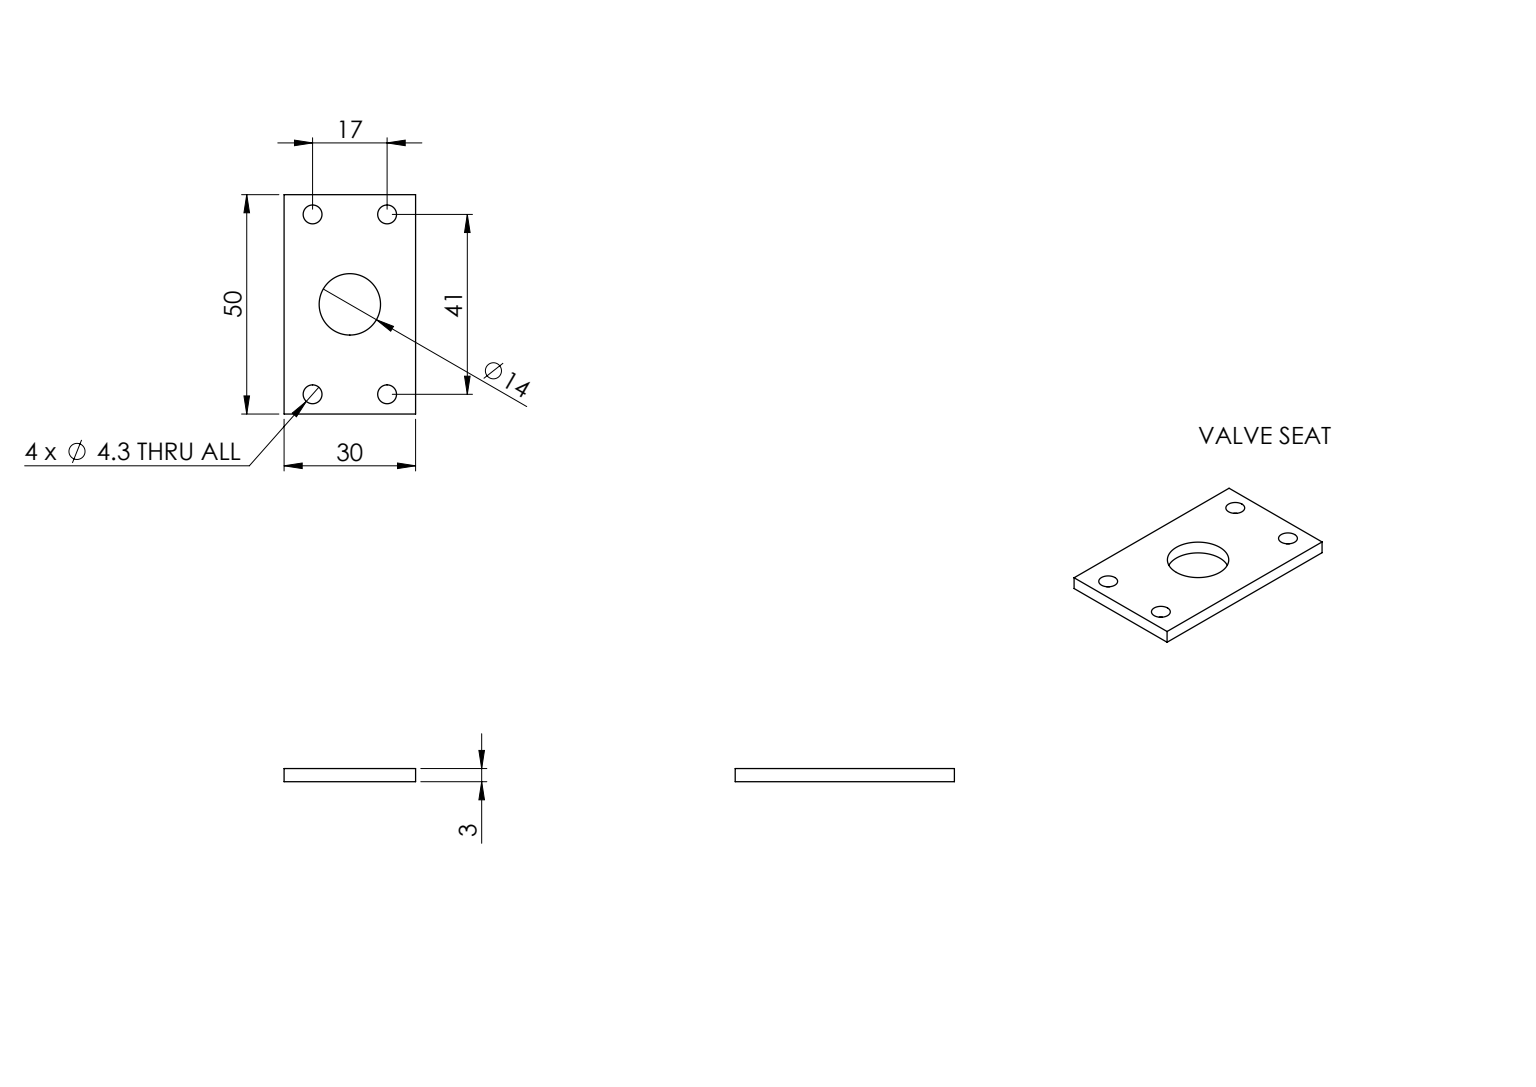
ISO-10303-21;
HEADER;
FILE_DESCRIPTION (('STEP AP214'),
    '1' );
FILE_NAME ('valve seat.step',
    '2026-10-25T16:39:07',
    ( '' ),
    ( '' ),
    'SwSTEP 2.0',
    'SolidWorks 2026',
    '' );
FILE_SCHEMA (( 'AUTOMOTIVE_DESIGN' ));
ENDSEC;

DATA;
#13=VERTEX_POINT ( 'NONE', #16013 ) ;
#121=CARTESIAN_POINT ( 'NONE',  ( 8.500000000000001776, 13.00000000000000178, -20.49999999999999645 ) ) ;
#128=DIRECTION ( 'NONE',  ( -1.000000000000000000, -0.000000000000000000, -0.000000000000000000 ) ) ;
#265=CARTESIAN_POINT ( 'NONE',  ( 8.673617379884035472E-15, 13.00000000000000178, 3.469446951953614189E-15 ) ) ;
#291=ORIENTED_EDGE ( 'NONE', *, *, #12084, .T. ) ;
#295=( NAMED_UNIT ( * ) PLANE_ANGLE_UNIT ( ) SI_UNIT ( $, .RADIAN. ) );
#319=EDGE_CURVE ( 'NONE', #18210, #10649, #7063, .T. ) ;
#321=LINE ( 'NONE', #17400, #16399 ) ;
#436=CARTESIAN_POINT ( 'NONE',  ( 14.99999999999999822, 13.00000000000000178, -25.00000000000000355 ) ) ;
#493=AXIS2_PLACEMENT_3D ( 'NONE', #9507, #8120, #16856 ) ;
#497=FACE_OUTER_BOUND ( 'NONE', #16040, .T. ) ;
#498=ORIENTED_EDGE ( 'NONE', *, *, #5184, .F. ) ;
#538=DIRECTION ( 'NONE',  ( -1.000000000000000000, 0.000000000000000000, 0.000000000000000000 ) ) ;
#543=AXIS2_PLACEMENT_3D ( 'NONE', #16285, #14984, #3573 ) ;
#557=( NAMED_UNIT ( * ) SI_UNIT ( $, .STERADIAN. ) SOLID_ANGLE_UNIT ( ) );
#636=FACE_OUTER_BOUND ( 'NONE', #10821, .T. ) ;
#646=VERTEX_POINT ( 'NONE', #1074 ) ;
#653=ORIENTED_EDGE ( 'NONE', *, *, #13216, .F. ) ;
#734=ADVANCED_FACE ( 'NONE', ( #5775 ), #14125, .F. ) ;
#775=EDGE_LOOP ( 'NONE', ( #10453, #6606, #13929, #968 ) ) ;
#797=DIRECTION ( 'NONE',  ( 0.000000000000000000, 0.000000000000000000, 1.000000000000000000 ) ) ;
#806=ORIENTED_EDGE ( 'NONE', *, *, #9638, .F. ) ;
#822=AXIS2_PLACEMENT_3D ( 'NONE', #16795, #15489, #1027 ) ;
#885=AXIS2_PLACEMENT_3D ( 'NONE', #7012, #8412, #13804 ) ;
#927=AXIS2_PLACEMENT_3D ( 'NONE', #1459, #7089, #2934 ) ;
#968=ORIENTED_EDGE ( 'NONE', *, *, #11920, .T. ) ;
#979=DIRECTION ( 'NONE',  ( -0.000000000000000000, -0.000000000000000000, 1.000000000000000000 ) ) ;
#991=VECTOR ( 'NONE', #7879, 1000.000000000000000 ) ;
#999=CARTESIAN_POINT ( 'NONE',  ( -15.00000000000000178, 13.00000000000000178, 24.99999999999999645 ) ) ;
#1027=DIRECTION ( 'NONE',  ( 0.000000000000000000, 0.000000000000000000, 1.000000000000000000 ) ) ;
#1074=CARTESIAN_POINT ( 'NONE',  ( 8.499999999999994671, 13.00000000000000178, 18.35000000000000142 ) ) ;
#1077=VECTOR ( 'NONE', #14132, 1000.000000000000000 ) ;
#1182=CARTESIAN_POINT ( 'NONE',  ( 8.500000000000001776, 10.00000000000000000, -20.49999999999999645 ) ) ;
#1189=CYLINDRICAL_SURFACE ( 'NONE', #927, 2.149999999999995470 ) ;
#1217=ORIENTED_EDGE ( 'NONE', *, *, #2834, .F. ) ;
#1266=ORIENTED_EDGE ( 'NONE', *, *, #2716, .F. ) ;
#1275=DIRECTION ( 'NONE',  ( -0.000000000000000000, 1.000000000000000000, -0.000000000000000000 ) ) ;
#1360=DIRECTION ( 'NONE',  ( 0.000000000000000000, 0.000000000000000000, 1.000000000000000000 ) ) ;
#1384=ADVANCED_FACE ( 'NONE', ( #11965 ), #2159, .F. ) ;
#1454=AXIS2_PLACEMENT_3D ( 'NONE', #1182, #11165, #2395 ) ;
#1459=CARTESIAN_POINT ( 'NONE',  ( 8.499999999999994671, 15.00000000000000178, 20.49999999999999645 ) ) ;
#1550=AXIS2_PLACEMENT_3D ( 'NONE', #5822, #8419, #10170 ) ;
#1564=CIRCLE ( 'NONE', #16681, 2.149999999999999023 ) ;
#1648=FACE_OUTER_BOUND ( 'NONE', #6847, .T. ) ;
#1684=DIRECTION ( 'NONE',  ( -0.000000000000000000, -0.000000000000000000, 1.000000000000000000 ) ) ;
#1737=CYLINDRICAL_SURFACE ( 'NONE', #18184, 2.149999999999995470 ) ;
#1770=ORIENTED_EDGE ( 'NONE', *, *, #6248, .F. ) ;
#1813=EDGE_LOOP ( 'NONE', ( #2295, #17707 ) ) ;
#1838=MECHANICAL_DESIGN_GEOMETRIC_PRESENTATION_REPRESENTATION('',(#15169),#7739);
#1880=FACE_OUTER_BOUND ( 'NONE', #2980, .T. ) ;
#1917=EDGE_CURVE ( 'NONE', #2431, #13322, #9840, .T. ) ;
#1959=VERTEX_POINT ( 'NONE', #6006 ) ;
#1975=DIRECTION ( 'NONE',  ( 0.000000000000000000, 0.000000000000000000, 1.000000000000000000 ) ) ;
#2030=ADVANCED_FACE ( 'NONE', ( #15844 ), #16037, .F. ) ;
#2053=VECTOR ( 'NONE', #4732, 1000.000000000000000 ) ;
#2080=PLANE ( 'NONE',  #12045 ) ;
#2099=EDGE_CURVE ( 'NONE', #13, #16617, #1564, .T. ) ;
#2103=FACE_BOUND ( 'NONE', #1813, .T. ) ;
#2159=PLANE ( 'NONE',  #10421 ) ;
#2184=EDGE_LOOP ( 'NONE', ( #18223, #5378, #6453, #10869 ) ) ;
#2195=FACE_BOUND ( 'NONE', #2494, .T. ) ;
#2204=VERTEX_POINT ( 'NONE', #17186 ) ;
#2206=CYLINDRICAL_SURFACE ( 'NONE', #8950, 2.149999999999995470 ) ;
#2208=DIRECTION ( 'NONE',  ( -0.000000000000000000, 1.000000000000000000, -0.000000000000000000 ) ) ;
#2217=PLANE ( 'NONE',  #16276 ) ;
#2218=MANIFOLD_SOLID_BREP ( 'M4 Clearance Hole1', #2906 ) ;
#2246=ORIENTED_EDGE ( 'NONE', *, *, #11807, .F. ) ;
#2254=LINE ( 'NONE', #9092, #991 ) ;
#2268=EDGE_LOOP ( 'NONE', ( #13436, #12204, #9696, #9451 ) ) ;
#2269=VERTEX_POINT ( 'NONE', #3262 ) ;
#2272=ORIENTED_EDGE ( 'NONE', *, *, #13752, .T. ) ;
#2295=ORIENTED_EDGE ( 'NONE', *, *, #15819, .F. ) ;
#2298=CIRCLE ( 'NONE', #9082, 2.149999999999999023 ) ;
#2306=ADVANCED_FACE ( 'NONE', ( #1880 ), #14577, .F. ) ;
#2314=VECTOR ( 'NONE', #15723, 1000.000000000000000 ) ;
#2375=CARTESIAN_POINT ( 'NONE',  ( 0.000000000000000000, 13.00000000000000178, 0.000000000000000000 ) ) ;
#2395=DIRECTION ( 'NONE',  ( 0.000000000000000000, 0.000000000000000000, 1.000000000000000000 ) ) ;
#2431=VERTEX_POINT ( 'NONE', #16518 ) ;
#2492=CARTESIAN_POINT ( 'NONE',  ( 8.673617379884035472E-15, 13.00000000000000178, 3.469446951953614189E-15 ) ) ;
#2494=EDGE_LOOP ( 'NONE', ( #9062, #15099 ) ) ;
#2539=ORIENTED_EDGE ( 'NONE', *, *, #17953, .T. ) ;
#2610=ORIENTED_EDGE ( 'NONE', *, *, #3037, .T. ) ;
#2617=VECTOR ( 'NONE', #12733, 1000.000000000000000 ) ;
#2619=EDGE_LOOP ( 'NONE', ( #9085, #6999 ) ) ;
#2630=ORIENTED_EDGE ( 'NONE', *, *, #4559, .F. ) ;
#2716=EDGE_CURVE ( 'NONE', #5029, #13163, #321, .T. ) ;
#2755=CARTESIAN_POINT ( 'NONE',  ( 8.673617379884035472E-15, 10.00000000000000000, -6.999999999999996447 ) ) ;
#2778=ORIENTED_EDGE ( 'NONE', *, *, #9638, .T. ) ;
#2780=CARTESIAN_POINT ( 'NONE',  ( -15.00000000000000178, 13.00000000000000178, 24.99999999999999645 ) ) ;
#2825=DIRECTION ( 'NONE',  ( 0.000000000000000000, 0.000000000000000000, -1.000000000000000000 ) ) ;
#2834=EDGE_CURVE ( 'NONE', #7772, #3408, #17185, .T. ) ;
#2855=CIRCLE ( 'NONE', #493, 2.149999999999995470 ) ;
#2896=VERTEX_POINT ( 'NONE', #11770 ) ;
#2906=CLOSED_SHELL ( 'NONE', ( #734, #2306, #10402, #14951, #12373, #4515, #10108, #15058, #1384, #7566, #10663, #2030, #4792, #17733, #3930, #18078 ) ) ;
#2923=DIRECTION ( 'NONE',  ( 1.000000000000000000, 0.000000000000000000, 0.000000000000000000 ) ) ;
#2934=DIRECTION ( 'NONE',  ( 0.000000000000000000, 0.000000000000000000, 1.000000000000000000 ) ) ;
#2980=EDGE_LOOP ( 'NONE', ( #16300, #15846, #10901, #18032 ) ) ;
#2998=DIRECTION ( 'NONE',  ( -0.000000000000000000, 1.000000000000000000, -0.000000000000000000 ) ) ;
#3037=EDGE_CURVE ( 'NONE', #2269, #2431, #8332, .T. ) ;
#3044=DIRECTION ( 'NONE',  ( 0.000000000000000000, 0.000000000000000000, 1.000000000000000000 ) ) ;
#3146=( NAMED_UNIT ( * ) SI_UNIT ( $, .STERADIAN. ) SOLID_ANGLE_UNIT ( ) );
#3155=ORIENTED_EDGE ( 'NONE', *, *, #15116, .F. ) ;
#3163=EDGE_CURVE ( 'NONE', #13322, #2431, #10104, .T. ) ;
#3233=DIRECTION ( 'NONE',  ( 0.000000000000000000, 0.000000000000000000, -1.000000000000000000 ) ) ;
#3262=CARTESIAN_POINT ( 'NONE',  ( -8.500000000000010658, 10.00000000000000000, 22.64999999999998437 ) ) ;
#3317=EDGE_LOOP ( 'NONE', ( #16483, #11941, #1266, #4428 ) ) ;
#3329=DIRECTION ( 'NONE',  ( -0.000000000000000000, -1.000000000000000000, -0.000000000000000000 ) ) ;
#3336=DIRECTION ( 'NONE',  ( 0.000000000000000000, 0.000000000000000000, -1.000000000000000000 ) ) ;
#3374=CARTESIAN_POINT ( 'NONE',  ( 8.673617379884035472E-15, 13.00000000000000178, 3.469446951953614189E-15 ) ) ;
#3408=VERTEX_POINT ( 'NONE', #6099 ) ;
#3460=CARTESIAN_POINT ( 'NONE',  ( -8.500000000000005329, 13.00000000000000178, -22.64999999999999147 ) ) ;
#3490=PRODUCT_CONTEXT ( 'NONE', #10071, 'mechanical' ) ;
#3549=CIRCLE ( 'NONE', #885, 7.000000000000000000 ) ;
#3573=DIRECTION ( 'NONE',  ( 0.000000000000000000, 0.000000000000000000, 1.000000000000000000 ) ) ;
#3624=DIRECTION ( 'NONE',  ( -0.000000000000000000, 1.000000000000000000, -0.000000000000000000 ) ) ;
#3641=CARTESIAN_POINT ( 'NONE',  ( -15.00000000000000178, 13.00000000000000178, 24.99999999999999645 ) ) ;
#3642=AXIS2_PLACEMENT_3D ( 'NONE', #16523, #10485, #16338 ) ;
#3668=FACE_OUTER_BOUND ( 'NONE', #14133, .T. ) ;
#3714=PLANE ( 'NONE',  #3642 ) ;
#3795=CARTESIAN_POINT ( 'NONE',  ( -8.500000000000010658, 15.00000000000000178, 22.64999999999998437 ) ) ;
#3870=ORIENTED_EDGE ( 'NONE', *, *, #1917, .T. ) ;
#3930=ADVANCED_FACE ( 'NONE', ( #9230 ), #2206, .F. ) ;
#3990=CIRCLE ( 'NONE', #12545, 2.149999999999995470 ) ;
#4020=CARTESIAN_POINT ( 'NONE',  ( 8.500000000000001776, 10.00000000000000000, -20.49999999999999645 ) ) ;
#4274=ORIENTED_EDGE ( 'NONE', *, *, #10452, .F. ) ;
#4275=ORIENTED_EDGE ( 'NONE', *, *, #13245, .F. ) ;
#4290=DIRECTION ( 'NONE',  ( 0.000000000000000000, 0.000000000000000000, 1.000000000000000000 ) ) ;
#4327=ORIENTED_EDGE ( 'NONE', *, *, #15402, .T. ) ;
#4416=VERTEX_POINT ( 'NONE', #17565 ) ;
#4428=ORIENTED_EDGE ( 'NONE', *, *, #16591, .T. ) ;
#4500=LINE ( 'NONE', #10140, #18114 ) ;
#4515=ADVANCED_FACE ( 'NONE', ( #17923, #10847, #13536, #4837, #6409, #7605 ), #3714, .T. ) ;
#4524=ORIENTED_EDGE ( 'NONE', *, *, #12834, .F. ) ;
#4559=EDGE_CURVE ( 'NONE', #2896, #7772, #2254, .T. ) ;
#4578=VERTEX_POINT ( 'NONE', #16141 ) ;
#4594=CARTESIAN_POINT ( 'NONE',  ( -8.500000000000010658, 15.00000000000000178, 20.49999999999998934 ) ) ;
#4626=ORIENTED_EDGE ( 'NONE', *, *, #14416, .F. ) ;
#4670=VECTOR ( 'NONE', #17689, 1000.000000000000000 ) ;
#4709=LINE ( 'NONE', #10072, #18017 ) ;
#4732=DIRECTION ( 'NONE',  ( -0.000000000000000000, -1.000000000000000000, -0.000000000000000000 ) ) ;
#4792=ADVANCED_FACE ( 'NONE', ( #12934 ), #1737, .F. ) ;
#4797=AXIS2_PLACEMENT_3D ( 'NONE', #17933, #16813, #10950 ) ;
#4837=FACE_OUTER_BOUND ( 'NONE', #16452, .T. ) ;
#4865=FACE_OUTER_BOUND ( 'NONE', #2268, .T. ) ;
#4889=CARTESIAN_POINT ( 'NONE',  ( 8.500000000000001776, 13.00000000000000178, -20.49999999999999645 ) ) ;
#4916=VECTOR ( 'NONE', #9948, 1000.000000000000000 ) ;
#4951=AXIS2_PLACEMENT_3D ( 'NONE', #4889, #15936, #3233 ) ;
#4963=DIRECTION ( 'NONE',  ( 0.000000000000000000, 0.000000000000000000, 1.000000000000000000 ) ) ;
#5029=VERTEX_POINT ( 'NONE', #436 ) ;
#5114=AXIS2_PLACEMENT_3D ( 'NONE', #16334, #3624, #16243 ) ;
#5122=VERTEX_POINT ( 'NONE', #17701 ) ;
#5158=DIRECTION ( 'NONE',  ( 0.000000000000000000, 0.000000000000000000, 1.000000000000000000 ) ) ;
#5184=EDGE_CURVE ( 'NONE', #13, #646, #14632, .T. ) ;
#5187=ORIENTED_EDGE ( 'NONE', *, *, #17953, .F. ) ;
#5202=ORIENTED_EDGE ( 'NONE', *, *, #5184, .T. ) ;
#5228=LINE ( 'NONE', #16563, #2617 ) ;
#5283=ORIENTED_EDGE ( 'NONE', *, *, #3163, .T. ) ;
#5306=SHAPE_REPRESENTATION ( 'valve seat', ( #16940 ), #7446 ) ;
#5327=AXIS2_PLACEMENT_3D ( 'NONE', #2780, #5541, #11549 ) ;
#5378=ORIENTED_EDGE ( 'NONE', *, *, #8416, .T. ) ;
#5461=CARTESIAN_POINT ( 'NONE',  ( -8.500000000000005329, 10.00000000000000000, -20.49999999999999645 ) ) ;
#5524=CARTESIAN_POINT ( 'NONE',  ( -8.500000000000005329, 15.00000000000000178, -18.35000000000000142 ) ) ;
#5541=DIRECTION ( 'NONE',  ( 1.000000000000000000, -0.000000000000000000, 0.000000000000000000 ) ) ;
#5573=AXIS2_PLACEMENT_3D ( 'NONE', #121, #9853, #2825 ) ;
#5601=DIRECTION ( 'NONE',  ( -0.000000000000000000, 1.000000000000000000, -0.000000000000000000 ) ) ;
#5638=VECTOR ( 'NONE', #14121, 1000.000000000000000 ) ;
#5664=VERTEX_POINT ( 'NONE', #13474 ) ;
#5697=CARTESIAN_POINT ( 'NONE',  ( -15.00000000000000178, 13.00000000000000178, 24.99999999999999645 ) ) ;
#5712=CARTESIAN_POINT ( 'NONE',  ( 14.99999999999999822, 10.00000000000000000, 24.99999999999999645 ) ) ;
#5715=MECHANICAL_DESIGN_GEOMETRIC_PRESENTATION_REPRESENTATION('',(#6603),#14001);
#5775=FACE_OUTER_BOUND ( 'NONE', #6105, .T. ) ;
#5822=CARTESIAN_POINT ( 'NONE',  ( -8.500000000000010658, 13.00000000000000178, 20.49999999999998934 ) ) ;
#5847=CIRCLE ( 'NONE', #16526, 2.149999999999995470 ) ;
#5861=CARTESIAN_POINT ( 'NONE',  ( -8.500000000000010658, 10.00000000000000000, 20.49999999999998934 ) ) ;
#6006=CARTESIAN_POINT ( 'NONE',  ( 8.500000000000001776, 10.00000000000000000, -22.64999999999999503 ) ) ;
#6014=VECTOR ( 'NONE', #6757, 1000.000000000000000 ) ;
#6049=LINE ( 'NONE', #6337, #6760 ) ;
#6083=VECTOR ( 'NONE', #2923, 1000.000000000000000 ) ;
#6092=ORIENTED_EDGE ( 'NONE', *, *, #2099, .T. ) ;
#6099=CARTESIAN_POINT ( 'NONE',  ( -15.00000000000000178, 10.00000000000000000, 24.99999999999999645 ) ) ;
#6105=EDGE_LOOP ( 'NONE', ( #13504, #17153, #806, #7661 ) ) ;
#6117=LINE ( 'NONE', #10281, #2053 ) ;
#6131=AXIS2_PLACEMENT_3D ( 'NONE', #17103, #2998, #17483 ) ;
#6187=LINE ( 'NONE', #13226, #12611 ) ;
#6204=EDGE_LOOP ( 'NONE', ( #6356, #2272 ) ) ;
#6207=EDGE_LOOP ( 'NONE', ( #498, #4275, #11171, #12765 ) ) ;
#6248=EDGE_CURVE ( 'NONE', #3408, #17590, #18338, .T. ) ;
#6274=COLOUR_RGB ( '',0.8941176470588234615, 0.8941176470588234615, 0.8941176470588234615 ) ;
#6275=CARTESIAN_POINT ( 'NONE',  ( -15.00000000000000178, 10.00000000000000000, -25.00000000000000355 ) ) ;
#6337=CARTESIAN_POINT ( 'NONE',  ( 8.500000000000001776, 15.00000000000000178, -22.64999999999999147 ) ) ;
#6356=ORIENTED_EDGE ( 'NONE', *, *, #13216, .T. ) ;
#6409=FACE_BOUND ( 'NONE', #2619, .T. ) ;
#6428=DIRECTION ( 'NONE',  ( 1.000000000000000000, 0.000000000000000000, 0.000000000000000000 ) ) ;
#6438=FACE_BOUND ( 'NONE', #9250, .T. ) ;
#6443=CARTESIAN_POINT ( 'NONE',  ( 14.99999999999999822, 13.00000000000000178, 24.99999999999999645 ) ) ;
#6453=ORIENTED_EDGE ( 'NONE', *, *, #13386, .T. ) ;
#6457=DIRECTION ( 'NONE',  ( 0.000000000000000000, 0.000000000000000000, 1.000000000000000000 ) ) ;
#6491=PRODUCT_DEFINITION_CONTEXT ( 'detailed design', #6987, 'design' ) ;
#6603=STYLED_ITEM('',(#18424),#2218);
#6606=ORIENTED_EDGE ( 'NONE', *, *, #16591, .F. ) ;
#6626=CARTESIAN_POINT ( 'NONE',  ( 14.99999999999999822, 13.00000000000000178, 24.99999999999999645 ) ) ;
#6687=VERTEX_POINT ( 'NONE', #15880 ) ;
#6757=DIRECTION ( 'NONE',  ( -0.000000000000000000, 1.000000000000000000, -0.000000000000000000 ) ) ;
#6760=VECTOR ( 'NONE', #17489, 1000.000000000000000 ) ;
#6811=EDGE_CURVE ( 'NONE', #5122, #4416, #12334, .T. ) ;
#6814=ORIENTED_EDGE ( 'NONE', *, *, #9269, .F. ) ;
#6847=EDGE_LOOP ( 'NONE', ( #9333, #4524, #12672, #13933 ) ) ;
#6902=ORIENTED_EDGE ( 'NONE', *, *, #3163, .F. ) ;
#6947=UNCERTAINTY_MEASURE_WITH_UNIT (LENGTH_MEASURE( 1.000000000000000082E-05 ), #10172, 'distance_accuracy_value', 'NONE');
#6987=APPLICATION_CONTEXT ( 'automotive_design' ) ;
#6999=ORIENTED_EDGE ( 'NONE', *, *, #14791, .T. ) ;
#7012=CARTESIAN_POINT ( 'NONE',  ( 8.673617379884035472E-15, 10.00000000000000000, 3.469446951953614189E-15 ) ) ;
#7034=ORIENTED_EDGE ( 'NONE', *, *, #11920, .F. ) ;
#7063=CIRCLE ( 'NONE', #17155, 2.149999999999995470 ) ;
#7089=DIRECTION ( 'NONE',  ( -0.000000000000000000, 1.000000000000000000, -0.000000000000000000 ) ) ;
#7097=DIRECTION ( 'NONE',  ( 0.000000000000000000, 0.000000000000000000, 1.000000000000000000 ) ) ;
#7115=EDGE_LOOP ( 'NONE', ( #4626, #3155, #16825, #10215 ) ) ;
#7132=AXIS2_PLACEMENT_3D ( 'NONE', #16380, #14811, #797 ) ;
#7396=SURFACE_STYLE_FILL_AREA ( #13055 ) ;
#7446=( GEOMETRIC_REPRESENTATION_CONTEXT ( 3 ) GLOBAL_UNCERTAINTY_ASSIGNED_CONTEXT ( ( #18290 ) ) GLOBAL_UNIT_ASSIGNED_CONTEXT ( ( #7674, #10364, #3146 ) ) REPRESENTATION_CONTEXT ( 'NONE', 'WORKASPACE' ) );
#7464=VERTEX_POINT ( 'NONE', #16696 ) ;
#7477=DIRECTION ( 'NONE',  ( 0.000000000000000000, 0.000000000000000000, -1.000000000000000000 ) ) ;
#7566=ADVANCED_FACE ( 'NONE', ( #1648 ), #10159, .F. ) ;
#7568=VECTOR ( 'NONE', #14280, 1000.000000000000000 ) ;
#7605=FACE_BOUND ( 'NONE', #15364, .T. ) ;
#7641=CYLINDRICAL_SURFACE ( 'NONE', #7132, 2.149999999999995470 ) ;
#7655=CYLINDRICAL_SURFACE ( 'NONE', #12104, 2.149999999999995470 ) ;
#7661=ORIENTED_EDGE ( 'NONE', *, *, #11348, .F. ) ;
#7674=( LENGTH_UNIT ( ) NAMED_UNIT ( * ) SI_UNIT ( .MILLI., .METRE. ) );
#7739=( GEOMETRIC_REPRESENTATION_CONTEXT ( 3 ) GLOBAL_UNCERTAINTY_ASSIGNED_CONTEXT ( ( #6947 ) ) GLOBAL_UNIT_ASSIGNED_CONTEXT ( ( #10172, #12958, #557 ) ) REPRESENTATION_CONTEXT ( 'NONE', 'WORKASPACE' ) );
#7772=VERTEX_POINT ( 'NONE', #6275 ) ;
#7778=AXIS2_PLACEMENT_3D ( 'NONE', #265, #3329, #15941 ) ;
#7805=CARTESIAN_POINT ( 'NONE',  ( -8.500000000000005329, 13.00000000000000178, -18.35000000000000142 ) ) ;
#7836=ADVANCED_BREP_SHAPE_REPRESENTATION ( '', ( #2218, #16940 ), #7446 ) ;
#7853=VERTEX_POINT ( 'NONE', #999 ) ;
#7872=CIRCLE ( 'NONE', #17070, 2.149999999999995470 ) ;
#7879=DIRECTION ( 'NONE',  ( -1.000000000000000000, -0.000000000000000000, -0.000000000000000000 ) ) ;
#7902=CIRCLE ( 'NONE', #10856, 2.149999999999995470 ) ;
#7932=DIRECTION ( 'NONE',  ( -0.000000000000000000, 1.000000000000000000, -0.000000000000000000 ) ) ;
#7960=DIRECTION ( 'NONE',  ( 0.000000000000000000, -1.000000000000000000, 0.000000000000000000 ) ) ;
#7969=EDGE_LOOP ( 'NONE', ( #9908, #15671 ) ) ;
#8120=DIRECTION ( 'NONE',  ( 0.000000000000000000, -1.000000000000000000, 0.000000000000000000 ) ) ;
#8124=VERTEX_POINT ( 'NONE', #2755 ) ;
#8145=CARTESIAN_POINT ( 'NONE',  ( -15.00000000000000178, 13.00000000000000178, -25.00000000000000355 ) ) ;
#8276=AXIS2_PLACEMENT_3D ( 'NONE', #11417, #17205, #8456 ) ;
#8332=LINE ( 'NONE', #3795, #6014 ) ;
#8405=ORIENTED_EDGE ( 'NONE', *, *, #11348, .T. ) ;
#8412=DIRECTION ( 'NONE',  ( 0.000000000000000000, 1.000000000000000000, 0.000000000000000000 ) ) ;
#8416=EDGE_CURVE ( 'NONE', #5122, #5664, #12783, .T. ) ;
#8419=DIRECTION ( 'NONE',  ( 0.000000000000000000, -1.000000000000000000, 0.000000000000000000 ) ) ;
#8456=DIRECTION ( 'NONE',  ( 0.000000000000000000, 0.000000000000000000, 1.000000000000000000 ) ) ;
#8686=SURFACE_SIDE_STYLE ('',( #7396 ) ) ;
#8706=EDGE_CURVE ( 'NONE', #11774, #646, #3990, .T. ) ;
#8707=CARTESIAN_POINT ( 'NONE',  ( -15.00000000000000178, 10.00000000000000000, 24.99999999999999645 ) ) ;
#8752=DIRECTION ( 'NONE',  ( -0.000000000000000000, 1.000000000000000000, -0.000000000000000000 ) ) ;
#8790=CIRCLE ( 'NONE', #822, 2.149999999999999023 ) ;
#8950=AXIS2_PLACEMENT_3D ( 'NONE', #10433, #11916, #4963 ) ;
#8965=LINE ( 'NONE', #15809, #1077 ) ;
#9024=CARTESIAN_POINT ( 'NONE',  ( 0.000000000000000000, 0.000000000000000000, 0.000000000000000000 ) ) ;
#9041=CARTESIAN_POINT ( 'NONE',  ( -8.500000000000005329, 13.00000000000000178, -20.49999999999999645 ) ) ;
#9058=DIRECTION ( 'NONE',  ( 0.000000000000000000, 0.000000000000000000, -1.000000000000000000 ) ) ;
#9062=ORIENTED_EDGE ( 'NONE', *, *, #8706, .T. ) ;
#9082=AXIS2_PLACEMENT_3D ( 'NONE', #4020, #12729, #4290 ) ;
#9085=ORIENTED_EDGE ( 'NONE', *, *, #10452, .T. ) ;
#9092=CARTESIAN_POINT ( 'NONE',  ( -15.00000000000000178, 10.00000000000000000, -25.00000000000000355 ) ) ;
#9151=CARTESIAN_POINT ( 'NONE',  ( 8.499999999999994671, 13.00000000000000178, 20.49999999999999645 ) ) ;
#9163=VECTOR ( 'NONE', #11369, 1000.000000000000000 ) ;
#9170=EDGE_CURVE ( 'NONE', #646, #11774, #7872, .T. ) ;
#9197=EDGE_CURVE ( 'NONE', #17590, #2896, #6187, .T. ) ;
#9230=FACE_OUTER_BOUND ( 'NONE', #7115, .T. ) ;
#9239=PRODUCT_DEFINITION_FORMATION_WITH_SPECIFIED_SOURCE ( 'ANY', '', #13293, .NOT_KNOWN. ) ;
#9250=EDGE_LOOP ( 'NONE', ( #3870, #5283 ) ) ;
#9265=EDGE_CURVE ( 'NONE', #13163, #7772, #8965, .T. ) ;
#9269=EDGE_CURVE ( 'NONE', #7853, #18081, #17031, .T. ) ;
#9288=DIRECTION ( 'NONE',  ( 0.000000000000000000, 0.000000000000000000, -1.000000000000000000 ) ) ;
#9333=ORIENTED_EDGE ( 'NONE', *, *, #2834, .T. ) ;
#9396=CARTESIAN_POINT ( 'NONE',  ( 8.500000000000001776, 15.00000000000000178, -18.35000000000000142 ) ) ;
#9451=ORIENTED_EDGE ( 'NONE', *, *, #9269, .T. ) ;
#9463=ORIENTED_EDGE ( 'NONE', *, *, #6248, .T. ) ;
#9507=CARTESIAN_POINT ( 'NONE',  ( -8.500000000000005329, 13.00000000000000178, -20.49999999999999645 ) ) ;
#9622=EDGE_LOOP ( 'NONE', ( #10639, #4327 ) ) ;
#9638=EDGE_CURVE ( 'NONE', #10649, #18210, #2855, .T. ) ;
#9696=ORIENTED_EDGE ( 'NONE', *, *, #10179, .T. ) ;
#9840=CIRCLE ( 'NONE', #18172, 2.149999999999995470 ) ;
#9853=DIRECTION ( 'NONE',  ( 0.000000000000000000, -1.000000000000000000, 0.000000000000000000 ) ) ;
#9874=FACE_OUTER_BOUND ( 'NONE', #6207, .T. ) ;
#9882=DIRECTION ( 'NONE',  ( -0.000000000000000000, 1.000000000000000000, -0.000000000000000000 ) ) ;
#9908=ORIENTED_EDGE ( 'NONE', *, *, #15116, .T. ) ;
#9924=VERTEX_POINT ( 'NONE', #16006 ) ;
#9948=DIRECTION ( 'NONE',  ( 1.000000000000000000, 0.000000000000000000, 0.000000000000000000 ) ) ;
#10023=CYLINDRICAL_SURFACE ( 'NONE', #6131, 2.149999999999995470 ) ;
#10071=APPLICATION_CONTEXT ( 'automotive_design' ) ;
#10072=CARTESIAN_POINT ( 'NONE',  ( 8.673617379884035472E-15, 13.00000000000000178, -6.999999999999996447 ) ) ;
#10104=CIRCLE ( 'NONE', #1550, 2.149999999999995470 ) ;
#10108=ADVANCED_FACE ( 'NONE', ( #13757, #16461, #2195, #6438, #4865, #2103 ), #14981, .F. ) ;
#10140=CARTESIAN_POINT ( 'NONE',  ( -8.500000000000010658, 15.00000000000000178, 18.34999999999999432 ) ) ;
#10159=PLANE ( 'NONE',  #5327 ) ;
#10170=DIRECTION ( 'NONE',  ( 0.000000000000000000, 0.000000000000000000, -1.000000000000000000 ) ) ;
#10172=( LENGTH_UNIT ( ) NAMED_UNIT ( * ) SI_UNIT ( .MILLI., .METRE. ) );
#10179=EDGE_CURVE ( 'NONE', #13163, #7853, #13659, .T. ) ;
#10191=( NAMED_UNIT ( * ) SI_UNIT ( $, .STERADIAN. ) SOLID_ANGLE_UNIT ( ) );
#10214=EDGE_CURVE ( 'NONE', #1959, #9924, #2298, .T. ) ;
#10215=ORIENTED_EDGE ( 'NONE', *, *, #10971, .F. ) ;
#10259=DIRECTION ( 'NONE',  ( 0.000000000000000000, 0.000000000000000000, 1.000000000000000000 ) ) ;
#10281=CARTESIAN_POINT ( 'NONE',  ( -15.00000000000000178, 13.00000000000000178, 24.99999999999999645 ) ) ;
#10363=CARTESIAN_POINT ( 'NONE',  ( -8.500000000000010658, 13.00000000000000178, 20.49999999999998934 ) ) ;
#10364=( NAMED_UNIT ( * ) PLANE_ANGLE_UNIT ( ) SI_UNIT ( $, .RADIAN. ) );
#10402=ADVANCED_FACE ( 'NONE', ( #15985 ), #10023, .F. ) ;
#10421=AXIS2_PLACEMENT_3D ( 'NONE', #16064, #1975, #13357 ) ;
#10433=CARTESIAN_POINT ( 'NONE',  ( 8.500000000000001776, 15.00000000000000178, -20.49999999999999645 ) ) ;
#10452=EDGE_CURVE ( 'NONE', #2269, #2204, #7902, .T. ) ;
#10453=ORIENTED_EDGE ( 'NONE', *, *, #9197, .T. ) ;
#10476=PRODUCT_DEFINITION_SHAPE ( 'NONE', 'NONE',  #16042 ) ;
#10485=DIRECTION ( 'NONE',  ( 0.000000000000000000, -1.000000000000000000, 0.000000000000000000 ) ) ;
#10515=DIRECTION ( 'NONE',  ( 0.000000000000000000, -0.000000000000000000, -1.000000000000000000 ) ) ;
#10540=EDGE_LOOP ( 'NONE', ( #17062, #5202, #13491, #18303 ) ) ;
#10591=CIRCLE ( 'NONE', #543, 7.000000000000000000 ) ;
#10609=LINE ( 'NONE', #6626, #16838 ) ;
#10639=ORIENTED_EDGE ( 'NONE', *, *, #11807, .T. ) ;
#10649=VERTEX_POINT ( 'NONE', #7805 ) ;
#10663=ADVANCED_FACE ( 'NONE', ( #12247 ), #2080, .F. ) ;
#10821=EDGE_LOOP ( 'NONE', ( #14972, #2539, #12113, #14563 ) ) ;
#10847=FACE_BOUND ( 'NONE', #7969, .T. ) ;
#10856=AXIS2_PLACEMENT_3D ( 'NONE', #5861, #11694, #17199 ) ;
#10869=ORIENTED_EDGE ( 'NONE', *, *, #15402, .F. ) ;
#10901=ORIENTED_EDGE ( 'NONE', *, *, #12084, .F. ) ;
#10929=DIRECTION ( 'NONE',  ( 0.000000000000000000, 0.000000000000000000, -1.000000000000000000 ) ) ;
#10950=DIRECTION ( 'NONE',  ( 0.000000000000000000, 0.000000000000000000, 1.000000000000000000 ) ) ;
#10971=EDGE_CURVE ( 'NONE', #7464, #16667, #18313, .T. ) ;
#11106=DIRECTION ( 'NONE',  ( -0.000000000000000000, 1.000000000000000000, -0.000000000000000000 ) ) ;
#11162=CIRCLE ( 'NONE', #15079, 2.149999999999995470 ) ;
#11165=DIRECTION ( 'NONE',  ( -0.000000000000000000, 1.000000000000000000, -0.000000000000000000 ) ) ;
#11171=ORIENTED_EDGE ( 'NONE', *, *, #15380, .T. ) ;
#11343=EDGE_CURVE ( 'NONE', #18081, #5029, #12751, .T. ) ;
#11348=EDGE_CURVE ( 'NONE', #4578, #10649, #15631, .T. ) ;
#11369=DIRECTION ( 'NONE',  ( -0.000000000000000000, 1.000000000000000000, -0.000000000000000000 ) ) ;
#11417=CARTESIAN_POINT ( 'NONE',  ( -8.500000000000005329, 15.00000000000000178, -20.49999999999999645 ) ) ;
#11418=DIRECTION ( 'NONE',  ( 0.000000000000000000, 0.000000000000000000, 1.000000000000000000 ) ) ;
#11435=CARTESIAN_POINT ( 'NONE',  ( 14.99999999999999822, 13.00000000000000178, 24.99999999999999645 ) ) ;
#11454=CARTESIAN_POINT ( 'NONE',  ( -8.500000000000010658, 10.00000000000000000, 20.49999999999998934 ) ) ;
#11476=CIRCLE ( 'NONE', #5573, 2.149999999999995470 ) ;
#11508=CARTESIAN_POINT ( 'NONE',  ( 8.499999999999994671, 10.00000000000000000, 22.64999999999999503 ) ) ;
#11549=DIRECTION ( 'NONE',  ( 0.000000000000000000, 0.000000000000000000, -1.000000000000000000 ) ) ;
#11550=DIRECTION ( 'NONE',  ( -0.000000000000000000, 1.000000000000000000, -0.000000000000000000 ) ) ;
#11655=CARTESIAN_POINT ( 'NONE',  ( 8.499999999999994671, 10.00000000000000000, 20.49999999999999645 ) ) ;
#11661=SHAPE_REPRESENTATION_RELATIONSHIP ( 'NONE' , 'NONE' ,  #5306, #7836 ) ;
#11694=DIRECTION ( 'NONE',  ( -0.000000000000000000, 1.000000000000000000, -0.000000000000000000 ) ) ;
#11770=CARTESIAN_POINT ( 'NONE',  ( 14.99999999999999822, 10.00000000000000000, -25.00000000000000355 ) ) ;
#11774=VERTEX_POINT ( 'NONE', #15164 ) ;
#11807=EDGE_CURVE ( 'NONE', #8124, #4416, #10591, .T. ) ;
#11812=CIRCLE ( 'NONE', #15480, 7.000000000000000000 ) ;
#11863=EDGE_CURVE ( 'NONE', #9924, #16667, #11995, .T. ) ;
#11916=DIRECTION ( 'NONE',  ( -0.000000000000000000, 1.000000000000000000, -0.000000000000000000 ) ) ;
#11920=EDGE_CURVE ( 'NONE', #18081, #17590, #10609, .T. ) ;
#11927=EDGE_CURVE ( 'NONE', #6687, #18210, #5228, .T. ) ;
#11929=CARTESIAN_POINT ( 'NONE',  ( -8.500000000000010658, 15.00000000000000178, 20.49999999999998934 ) ) ;
#11941=ORIENTED_EDGE ( 'NONE', *, *, #9265, .F. ) ;
#11965=FACE_OUTER_BOUND ( 'NONE', #3317, .T. ) ;
#11977=DIRECTION ( 'NONE',  ( -1.000000000000000000, 0.000000000000000000, -0.000000000000000000 ) ) ;
#11995=LINE ( 'NONE', #9396, #4670 ) ;
#12037=ORIENTED_EDGE ( 'NONE', *, *, #6811, .T. ) ;
#12045=AXIS2_PLACEMENT_3D ( 'NONE', #3641, #9288, #11977 ) ;
#12084=EDGE_CURVE ( 'NONE', #16667, #7464, #11476, .T. ) ;
#12104=AXIS2_PLACEMENT_3D ( 'NONE', #11929, #7932, #5158 ) ;
#12113=ORIENTED_EDGE ( 'NONE', *, *, #1917, .F. ) ;
#12118=ORIENTED_EDGE ( 'NONE', *, *, #10971, .T. ) ;
#12177=DIRECTION ( 'NONE',  ( 0.000000000000000000, -1.000000000000000000, 0.000000000000000000 ) ) ;
#12204=ORIENTED_EDGE ( 'NONE', *, *, #2716, .T. ) ;
#12247=FACE_OUTER_BOUND ( 'NONE', #13076, .T. ) ;
#12271=DIRECTION ( 'NONE',  ( -0.000000000000000000, -1.000000000000000000, -0.000000000000000000 ) ) ;
#12334=LINE ( 'NONE', #13064, #7568 ) ;
#12373=ADVANCED_FACE ( 'NONE', ( #497 ), #14693, .F. ) ;
#12425=ORIENTED_EDGE ( 'NONE', *, *, #319, .F. ) ;
#12545=AXIS2_PLACEMENT_3D ( 'NONE', #16700, #7960, #10929 ) ;
#12590=CARTESIAN_POINT ( 'NONE',  ( -8.500000000000010658, 13.00000000000000178, 18.34999999999999432 ) ) ;
#12611=VECTOR ( 'NONE', #9058, 1000.000000000000000 ) ;
#12672=ORIENTED_EDGE ( 'NONE', *, *, #10179, .F. ) ;
#12677=AXIS2_PLACEMENT_3D ( 'NONE', #3374, #16265, #17765 ) ;
#12729=DIRECTION ( 'NONE',  ( -0.000000000000000000, 1.000000000000000000, -0.000000000000000000 ) ) ;
#12733=DIRECTION ( 'NONE',  ( -0.000000000000000000, 1.000000000000000000, -0.000000000000000000 ) ) ;
#12751=LINE ( 'NONE', #11435, #2314 ) ;
#12765=ORIENTED_EDGE ( 'NONE', *, *, #9170, .F. ) ;
#12771=LINE ( 'NONE', #16881, #9163 ) ;
#12783=CIRCLE ( 'NONE', #4797, 7.000000000000000000 ) ;
#12797=ORIENTED_EDGE ( 'NONE', *, *, #9197, .F. ) ;
#12834=EDGE_CURVE ( 'NONE', #7853, #3408, #6117, .T. ) ;
#12934=FACE_OUTER_BOUND ( 'NONE', #17644, .T. ) ;
#12958=( NAMED_UNIT ( * ) PLANE_ANGLE_UNIT ( ) SI_UNIT ( $, .RADIAN. ) );
#12980=( LENGTH_UNIT ( ) NAMED_UNIT ( * ) SI_UNIT ( .MILLI., .METRE. ) );
#13055=FILL_AREA_STYLE ('',( #15755 ) ) ;
#13064=CARTESIAN_POINT ( 'NONE',  ( 9.530870139287183087E-15, 13.00000000000000178, 7.000000000000003553 ) ) ;
#13076=EDGE_LOOP ( 'NONE', ( #9463, #7034, #6814, #16578 ) ) ;
#13091=CARTESIAN_POINT ( 'NONE',  ( 14.99999999999999822, 13.00000000000000178, -25.00000000000000355 ) ) ;
#13163=VERTEX_POINT ( 'NONE', #8145 ) ;
#13216=EDGE_CURVE ( 'NONE', #4578, #6687, #11162, .T. ) ;
#13226=CARTESIAN_POINT ( 'NONE',  ( 14.99999999999999822, 10.00000000000000000, 24.99999999999999645 ) ) ;
#13239=SURFACE_STYLE_USAGE ( .BOTH. , #8686 ) ;
#13245=EDGE_CURVE ( 'NONE', #16617, #13, #8790, .T. ) ;
#13293=PRODUCT ( 'valve seat', 'valve seat', '', ( #3490 ) ) ;
#13322=VERTEX_POINT ( 'NONE', #12590 ) ;
#13357=DIRECTION ( 'NONE',  ( 1.000000000000000000, 0.000000000000000000, -0.000000000000000000 ) ) ;
#13386=EDGE_CURVE ( 'NONE', #5664, #8124, #4709, .T. ) ;
#13391=CARTESIAN_POINT ( 'NONE',  ( -15.00000000000000178, 13.00000000000000178, 24.99999999999999645 ) ) ;
#13436=ORIENTED_EDGE ( 'NONE', *, *, #11343, .T. ) ;
#13474=CARTESIAN_POINT ( 'NONE',  ( 8.673617379884035472E-15, 13.00000000000000178, -6.999999999999996447 ) ) ;
#13491=ORIENTED_EDGE ( 'NONE', *, *, #8706, .F. ) ;
#13504=ORIENTED_EDGE ( 'NONE', *, *, #13752, .F. ) ;
#13536=FACE_BOUND ( 'NONE', #9622, .T. ) ;
#13557=DIRECTION ( 'NONE',  ( 0.000000000000000000, 0.000000000000000000, 1.000000000000000000 ) ) ;
#13659=LINE ( 'NONE', #13391, #16206 ) ;
#13752=EDGE_CURVE ( 'NONE', #6687, #4578, #5847, .T. ) ;
#13757=FACE_BOUND ( 'NONE', #17327, .T. ) ;
#13804=DIRECTION ( 'NONE',  ( 0.000000000000000000, 0.000000000000000000, 1.000000000000000000 ) ) ;
#13928=ORIENTED_EDGE ( 'NONE', *, *, #319, .T. ) ;
#13929=ORIENTED_EDGE ( 'NONE', *, *, #11343, .F. ) ;
#13933=ORIENTED_EDGE ( 'NONE', *, *, #9265, .T. ) ;
#14001=( GEOMETRIC_REPRESENTATION_CONTEXT ( 3 ) GLOBAL_UNCERTAINTY_ASSIGNED_CONTEXT ( ( #15289 ) ) GLOBAL_UNIT_ASSIGNED_CONTEXT ( ( #12980, #295, #10191 ) ) REPRESENTATION_CONTEXT ( 'NONE', 'WORKASPACE' ) );
#14121=DIRECTION ( 'NONE',  ( -0.000000000000000000, -1.000000000000000000, -0.000000000000000000 ) ) ;
#14125=CYLINDRICAL_SURFACE ( 'NONE', #8276, 2.149999999999995470 ) ;
#14126=CARTESIAN_POINT ( 'NONE',  ( -8.500000000000005329, 10.00000000000000000, -20.49999999999999645 ) ) ;
#14132=DIRECTION ( 'NONE',  ( -0.000000000000000000, -1.000000000000000000, -0.000000000000000000 ) ) ;
#14133=EDGE_LOOP ( 'NONE', ( #17444, #653, #8405, #12425 ) ) ;
#14134=CARTESIAN_POINT ( 'NONE',  ( -15.00000000000000178, 10.00000000000000000, 24.99999999999999645 ) ) ;
#14280=DIRECTION ( 'NONE',  ( -0.000000000000000000, -1.000000000000000000, -0.000000000000000000 ) ) ;
#14363=PRESENTATION_STYLE_ASSIGNMENT (( #13239 ) ) ;
#14416=EDGE_CURVE ( 'NONE', #1959, #7464, #6049, .T. ) ;
#14563=ORIENTED_EDGE ( 'NONE', *, *, #3037, .F. ) ;
#14577=CYLINDRICAL_SURFACE ( 'NONE', #5114, 2.149999999999995470 ) ;
#14632=LINE ( 'NONE', #14917, #16397 ) ;
#14693=CYLINDRICAL_SURFACE ( 'NONE', #12677, 7.000000000000000000 ) ;
#14791=EDGE_CURVE ( 'NONE', #2204, #2269, #17162, .T. ) ;
#14811=DIRECTION ( 'NONE',  ( -0.000000000000000000, 1.000000000000000000, -0.000000000000000000 ) ) ;
#14907=DIRECTION ( 'NONE',  ( 0.000000000000000000, 0.000000000000000000, -1.000000000000000000 ) ) ;
#14917=CARTESIAN_POINT ( 'NONE',  ( 8.499999999999994671, 15.00000000000000178, 18.35000000000000142 ) ) ;
#14924=FACE_OUTER_BOUND ( 'NONE', #775, .T. ) ;
#14951=ADVANCED_FACE ( 'NONE', ( #636 ), #7655, .F. ) ;
#14972=ORIENTED_EDGE ( 'NONE', *, *, #14791, .F. ) ;
#14981=PLANE ( 'NONE',  #15029 ) ;
#14984=DIRECTION ( 'NONE',  ( 0.000000000000000000, 1.000000000000000000, 0.000000000000000000 ) ) ;
#15005=CARTESIAN_POINT ( 'NONE',  ( 14.99999999999999822, 13.00000000000000178, 24.99999999999999645 ) ) ;
#15029=AXIS2_PLACEMENT_3D ( 'NONE', #2375, #12177, #10515 ) ;
#15058=ADVANCED_FACE ( 'NONE', ( #14924 ), #2217, .F. ) ;
#15077=AXIS2_PLACEMENT_3D ( 'NONE', #11454, #11550, #3044 ) ;
#15079=AXIS2_PLACEMENT_3D ( 'NONE', #5461, #11106, #16886 ) ;
#15099=ORIENTED_EDGE ( 'NONE', *, *, #9170, .T. ) ;
#15116=EDGE_CURVE ( 'NONE', #9924, #1959, #16567, .T. ) ;
#15164=CARTESIAN_POINT ( 'NONE',  ( 8.499999999999994671, 13.00000000000000178, 22.64999999999999147 ) ) ;
#15169=STYLED_ITEM ( 'NONE', ( #14363 ), #7836 ) ;
#15177=VECTOR ( 'NONE', #1684, 1000.000000000000000 ) ;
#15289=UNCERTAINTY_MEASURE_WITH_UNIT (LENGTH_MEASURE( 1.000000000000000082E-05 ), #12980, 'distance_accuracy_value', 'NONE');
#15364=EDGE_LOOP ( 'NONE', ( #15847, #6092 ) ) ;
#15371=DIRECTION ( 'NONE',  ( 0.000000000000000000, 1.000000000000000000, 0.000000000000000000 ) ) ;
#15380=EDGE_CURVE ( 'NONE', #16617, #11774, #12771, .T. ) ;
#15402=EDGE_CURVE ( 'NONE', #4416, #8124, #3549, .T. ) ;
#15480=AXIS2_PLACEMENT_3D ( 'NONE', #2492, #15371, #1360 ) ;
#15489=DIRECTION ( 'NONE',  ( -0.000000000000000000, 1.000000000000000000, -0.000000000000000000 ) ) ;
#15566=DIRECTION ( 'NONE',  ( -0.000000000000000000, -1.000000000000000000, -0.000000000000000000 ) ) ;
#15631=LINE ( 'NONE', #5524, #17424 ) ;
#15671=ORIENTED_EDGE ( 'NONE', *, *, #10214, .T. ) ;
#15723=DIRECTION ( 'NONE',  ( 0.000000000000000000, 0.000000000000000000, -1.000000000000000000 ) ) ;
#15755=FILL_AREA_STYLE_COLOUR ( '', #6274 ) ;
#15798=CARTESIAN_POINT ( 'NONE',  ( 8.500000000000001776, 13.00000000000000178, -18.35000000000000142 ) ) ;
#15809=CARTESIAN_POINT ( 'NONE',  ( -15.00000000000000178, 13.00000000000000178, -25.00000000000000355 ) ) ;
#15819=EDGE_CURVE ( 'NONE', #5664, #5122, #11812, .T. ) ;
#15844=FACE_OUTER_BOUND ( 'NONE', #2184, .T. ) ;
#15846=ORIENTED_EDGE ( 'NONE', *, *, #14416, .T. ) ;
#15847=ORIENTED_EDGE ( 'NONE', *, *, #13245, .T. ) ;
#15880=CARTESIAN_POINT ( 'NONE',  ( -8.500000000000005329, 10.00000000000000000, -22.64999999999999147 ) ) ;
#15936=DIRECTION ( 'NONE',  ( 0.000000000000000000, -1.000000000000000000, 0.000000000000000000 ) ) ;
#15941=DIRECTION ( 'NONE',  ( 0.000000000000000000, 0.000000000000000000, -1.000000000000000000 ) ) ;
#15985=FACE_OUTER_BOUND ( 'NONE', #10540, .T. ) ;
#16006=CARTESIAN_POINT ( 'NONE',  ( 8.500000000000001776, 10.00000000000000000, -18.34999999999999787 ) ) ;
#16011=DIRECTION ( 'NONE',  ( 0.000000000000000000, -1.000000000000000000, 0.000000000000000000 ) ) ;
#16013=CARTESIAN_POINT ( 'NONE',  ( 8.499999999999994671, 10.00000000000000000, 18.34999999999999787 ) ) ;
#16037=CYLINDRICAL_SURFACE ( 'NONE', #7778, 7.000000000000000000 ) ;
#16040=EDGE_LOOP ( 'NONE', ( #16296, #12037, #2246, #16344 ) ) ;
#16042=PRODUCT_DEFINITION ( 'UNKNOWN', '', #9239, #6491 ) ;
#16043=DIRECTION ( 'NONE',  ( 0.000000000000000000, -1.000000000000000000, 0.000000000000000000 ) ) ;
#16064=CARTESIAN_POINT ( 'NONE',  ( -15.00000000000000178, 13.00000000000000178, -25.00000000000000355 ) ) ;
#16141=CARTESIAN_POINT ( 'NONE',  ( -8.500000000000005329, 10.00000000000000000, -18.35000000000000142 ) ) ;
#16206=VECTOR ( 'NONE', #979, 1000.000000000000000 ) ;
#16243=DIRECTION ( 'NONE',  ( 0.000000000000000000, 0.000000000000000000, 1.000000000000000000 ) ) ;
#16265=DIRECTION ( 'NONE',  ( -0.000000000000000000, -1.000000000000000000, -0.000000000000000000 ) ) ;
#16276=AXIS2_PLACEMENT_3D ( 'NONE', #15005, #538, #6457 ) ;
#16285=CARTESIAN_POINT ( 'NONE',  ( 8.673617379884035472E-15, 10.00000000000000000, 3.469446951953614189E-15 ) ) ;
#16296=ORIENTED_EDGE ( 'NONE', *, *, #15819, .T. ) ;
#16300=ORIENTED_EDGE ( 'NONE', *, *, #10214, .F. ) ;
#16305=DIRECTION ( 'NONE',  ( 0.000000000000000000, -1.000000000000000000, 0.000000000000000000 ) ) ;
#16334=CARTESIAN_POINT ( 'NONE',  ( 8.500000000000001776, 15.00000000000000178, -20.49999999999999645 ) ) ;
#16338=DIRECTION ( 'NONE',  ( 0.000000000000000000, -0.000000000000000000, -1.000000000000000000 ) ) ;
#16344=ORIENTED_EDGE ( 'NONE', *, *, #13386, .F. ) ;
#16380=CARTESIAN_POINT ( 'NONE',  ( -8.500000000000005329, 15.00000000000000178, -20.49999999999999645 ) ) ;
#16397=VECTOR ( 'NONE', #2208, 1000.000000000000000 ) ;
#16399=VECTOR ( 'NONE', #128, 1000.000000000000000 ) ;
#16452=EDGE_LOOP ( 'NONE', ( #12797, #1770, #1217, #2630 ) ) ;
#16461=FACE_BOUND ( 'NONE', #18009, .T. ) ;
#16483=ORIENTED_EDGE ( 'NONE', *, *, #4559, .T. ) ;
#16518=CARTESIAN_POINT ( 'NONE',  ( -8.500000000000010658, 13.00000000000000178, 22.64999999999998437 ) ) ;
#16523=CARTESIAN_POINT ( 'NONE',  ( 0.000000000000000000, 10.00000000000000000, 0.000000000000000000 ) ) ;
#16526=AXIS2_PLACEMENT_3D ( 'NONE', #14126, #5601, #11418 ) ;
#16563=CARTESIAN_POINT ( 'NONE',  ( -8.500000000000005329, 15.00000000000000178, -22.64999999999999147 ) ) ;
#16567=CIRCLE ( 'NONE', #1454, 2.149999999999999023 ) ;
#16578=ORIENTED_EDGE ( 'NONE', *, *, #12834, .T. ) ;
#16591=EDGE_CURVE ( 'NONE', #5029, #2896, #17201, .T. ) ;
#16617=VERTEX_POINT ( 'NONE', #11508 ) ;
#16667=VERTEX_POINT ( 'NONE', #15798 ) ;
#16681=AXIS2_PLACEMENT_3D ( 'NONE', #11655, #17349, #10259 ) ;
#16696=CARTESIAN_POINT ( 'NONE',  ( 8.500000000000001776, 13.00000000000000178, -22.64999999999999147 ) ) ;
#16700=CARTESIAN_POINT ( 'NONE',  ( 8.499999999999994671, 13.00000000000000178, 20.49999999999999645 ) ) ;
#16795=CARTESIAN_POINT ( 'NONE',  ( 8.499999999999994671, 10.00000000000000000, 20.49999999999999645 ) ) ;
#16813=DIRECTION ( 'NONE',  ( 0.000000000000000000, 1.000000000000000000, 0.000000000000000000 ) ) ;
#16825=ORIENTED_EDGE ( 'NONE', *, *, #11863, .T. ) ;
#16838=VECTOR ( 'NONE', #12271, 1000.000000000000000 ) ;
#16856=DIRECTION ( 'NONE',  ( 0.000000000000000000, 0.000000000000000000, -1.000000000000000000 ) ) ;
#16881=CARTESIAN_POINT ( 'NONE',  ( 8.499999999999994671, 15.00000000000000178, 22.64999999999999147 ) ) ;
#16886=DIRECTION ( 'NONE',  ( 0.000000000000000000, 0.000000000000000000, 1.000000000000000000 ) ) ;
#16940=AXIS2_PLACEMENT_3D ( 'NONE', #9024, #13557, #6428 ) ;
#17031=LINE ( 'NONE', #5697, #4916 ) ;
#17062=ORIENTED_EDGE ( 'NONE', *, *, #2099, .F. ) ;
#17070=AXIS2_PLACEMENT_3D ( 'NONE', #9151, #16305, #7477 ) ;
#17103=CARTESIAN_POINT ( 'NONE',  ( 8.499999999999994671, 15.00000000000000178, 20.49999999999999645 ) ) ;
#17153=ORIENTED_EDGE ( 'NONE', *, *, #11927, .T. ) ;
#17155=AXIS2_PLACEMENT_3D ( 'NONE', #9041, #16011, #14907 ) ;
#17162=CIRCLE ( 'NONE', #15077, 2.149999999999995470 ) ;
#17185=LINE ( 'NONE', #8707, #15177 ) ;
#17186=CARTESIAN_POINT ( 'NONE',  ( -8.500000000000010658, 10.00000000000000000, 18.34999999999999432 ) ) ;
#17199=DIRECTION ( 'NONE',  ( 0.000000000000000000, 0.000000000000000000, 1.000000000000000000 ) ) ;
#17201=LINE ( 'NONE', #13091, #5638 ) ;
#17205=DIRECTION ( 'NONE',  ( -0.000000000000000000, 1.000000000000000000, -0.000000000000000000 ) ) ;
#17327=EDGE_LOOP ( 'NONE', ( #2778, #13928 ) ) ;
#17349=DIRECTION ( 'NONE',  ( -0.000000000000000000, 1.000000000000000000, -0.000000000000000000 ) ) ;
#17400=CARTESIAN_POINT ( 'NONE',  ( -15.00000000000000178, 13.00000000000000178, -25.00000000000000355 ) ) ;
#17424=VECTOR ( 'NONE', #1275, 1000.000000000000000 ) ;
#17444=ORIENTED_EDGE ( 'NONE', *, *, #11927, .F. ) ;
#17483=DIRECTION ( 'NONE',  ( 0.000000000000000000, 0.000000000000000000, 1.000000000000000000 ) ) ;
#17489=DIRECTION ( 'NONE',  ( -0.000000000000000000, 1.000000000000000000, -0.000000000000000000 ) ) ;
#17565=CARTESIAN_POINT ( 'NONE',  ( 9.530870139287183087E-15, 10.00000000000000000, 7.000000000000003553 ) ) ;
#17590=VERTEX_POINT ( 'NONE', #5712 ) ;
#17644=EDGE_LOOP ( 'NONE', ( #5187, #4274, #2610, #6902 ) ) ;
#17689=DIRECTION ( 'NONE',  ( -0.000000000000000000, 1.000000000000000000, -0.000000000000000000 ) ) ;
#17701=CARTESIAN_POINT ( 'NONE',  ( 9.530870139287183087E-15, 13.00000000000000178, 7.000000000000003553 ) ) ;
#17707=ORIENTED_EDGE ( 'NONE', *, *, #8416, .F. ) ;
#17733=ADVANCED_FACE ( 'NONE', ( #9874 ), #1189, .F. ) ;
#17765=DIRECTION ( 'NONE',  ( 0.000000000000000000, 0.000000000000000000, -1.000000000000000000 ) ) ;
#17923=FACE_BOUND ( 'NONE', #6204, .T. ) ;
#17933=CARTESIAN_POINT ( 'NONE',  ( 8.673617379884035472E-15, 13.00000000000000178, 3.469446951953614189E-15 ) ) ;
#17953=EDGE_CURVE ( 'NONE', #2204, #13322, #4500, .T. ) ;
#17969=SHAPE_DEFINITION_REPRESENTATION ( #10476, #5306 ) ;
#18009=EDGE_LOOP ( 'NONE', ( #291, #12118 ) ) ;
#18017=VECTOR ( 'NONE', #15566, 1000.000000000000000 ) ;
#18032=ORIENTED_EDGE ( 'NONE', *, *, #11863, .F. ) ;
#18078=ADVANCED_FACE ( 'NONE', ( #3668 ), #7641, .F. ) ;
#18081=VERTEX_POINT ( 'NONE', #6443 ) ;
#18114=VECTOR ( 'NONE', #8752, 1000.000000000000000 ) ;
#18172=AXIS2_PLACEMENT_3D ( 'NONE', #10363, #16043, #3336 ) ;
#18184=AXIS2_PLACEMENT_3D ( 'NONE', #4594, #9882, #7097 ) ;
#18210=VERTEX_POINT ( 'NONE', #3460 ) ;
#18223=ORIENTED_EDGE ( 'NONE', *, *, #6811, .F. ) ;
#18290=UNCERTAINTY_MEASURE_WITH_UNIT (LENGTH_MEASURE( 1.000000000000000082E-05 ), #7674, 'distance_accuracy_value', 'NONE');
#18303=ORIENTED_EDGE ( 'NONE', *, *, #15380, .F. ) ;
#18313=CIRCLE ( 'NONE', #4951, 2.149999999999995470 ) ;
#18338=LINE ( 'NONE', #14134, #6083 ) ;
#18418=COLOUR_RGB('Off White',0.89,0.88,0.83);
#18419=FILL_AREA_STYLE_COLOUR('',#18418);
#18420=FILL_AREA_STYLE('',(#18419));
#18421=SURFACE_STYLE_FILL_AREA(#18420);
#18422=SURFACE_SIDE_STYLE('',(#18421));
#18423=SURFACE_STYLE_USAGE(.BOTH.,#18422);
#18424=PRESENTATION_STYLE_ASSIGNMENT((#18423));
ENDSEC;
END-ISO-10303-21;
